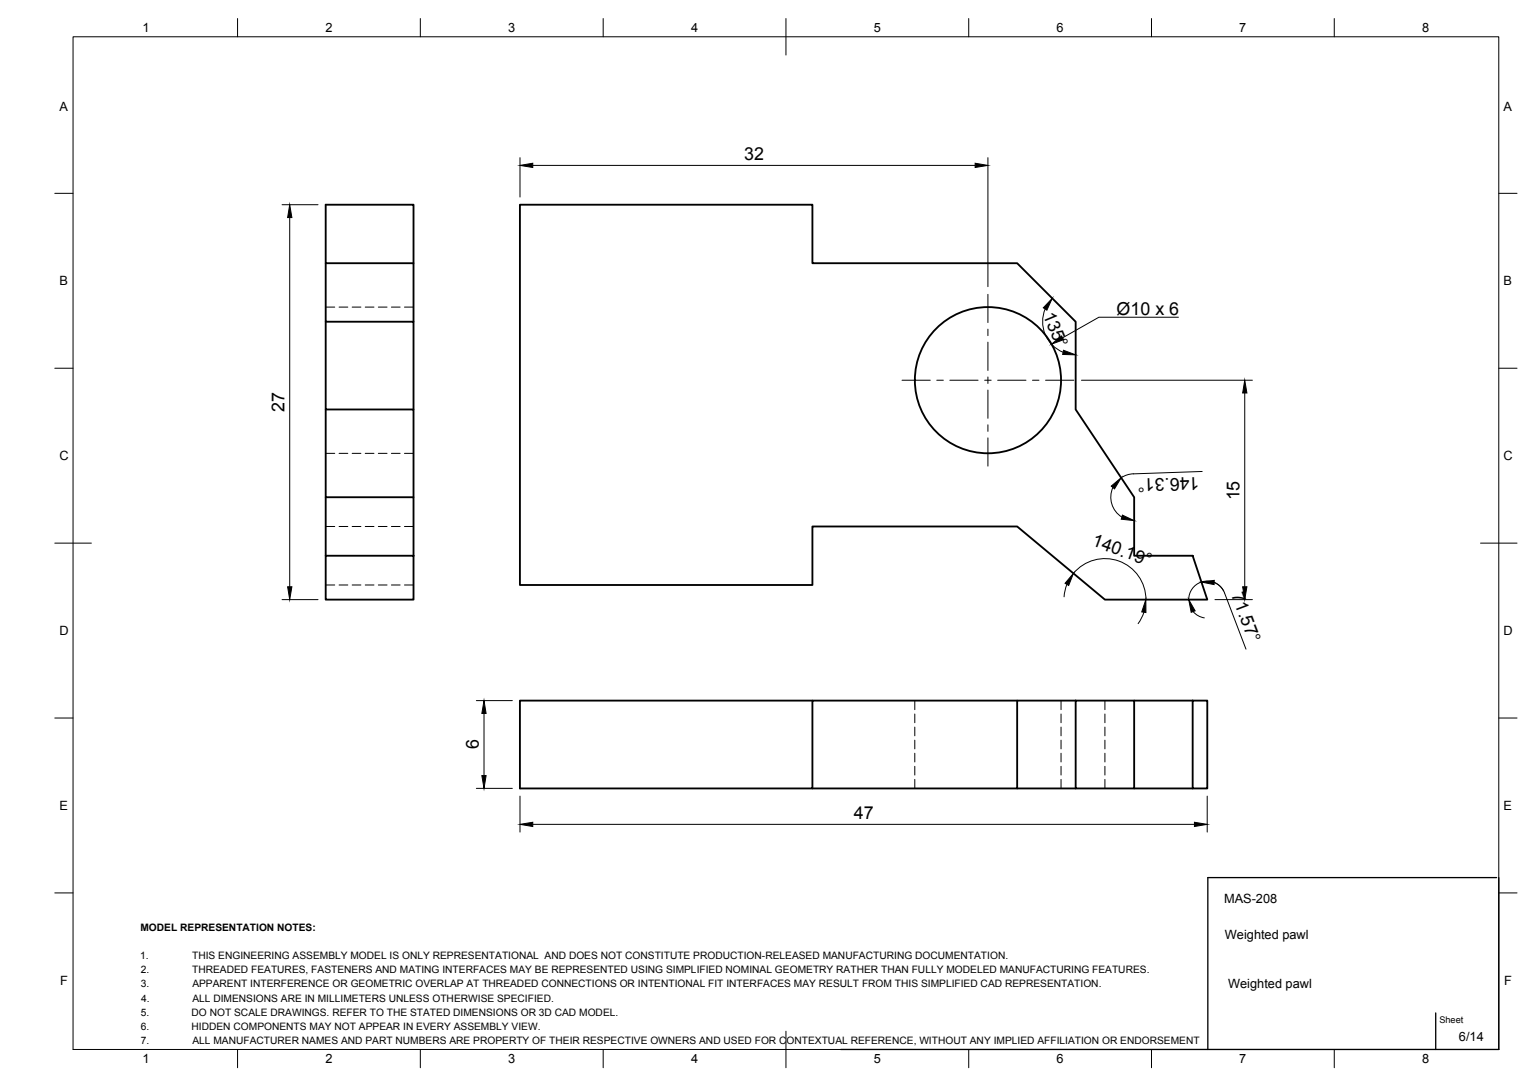
ISO-10303-21;
HEADER;
/* Generated by software containing ST-Developer
 * from STEP Tools, Inc. (www.steptools.com) 
 */

FILE_DESCRIPTION(
/* description */ ('Independent vertical20-tooth ratchet advance with repeated integral-c
ounterweight gravity pawls, swinging drive lever, bronze sleeves and f
ully retained axle stacks.18degpertooth. Native revolutes; geometric c
ycle checking rather than automatic contact/rolling dynamics. Gravity 
closing checked from actual pawl center of mass. Backplate/foot suppor
ts unit. Fits, torque, holding force, wear and life unassigned.'),
/* implementation_level */ '2;1');

FILE_NAME(
/* name */ 'Weighted pawl.step',
/* time_stamp */ '2026-11-09T06:25:53-08:00',
/* author */ (''),
/* organization */ (''),
/* preprocessor_version */ 'ST-DEVELOPER v20.2',
/* originating_system */ 'Autodesk Translation Framework v15.17.0.0',
/* authorisation */ '');

FILE_SCHEMA (('AUTOMOTIVE_DESIGN { 1 0 10303 214 3 1 1 }'));
ENDSEC;

DATA;
#10=MECHANICAL_DESIGN_GEOMETRIC_PRESENTATION_REPRESENTATION('',(#130),#4643);
#102=SHAPE_REPRESENTATION_RELATIONSHIP('SRR','None',#4707,#116);
#116=ADVANCED_BREP_SHAPE_REPRESENTATION('',(#144),#4636);
#130=STYLED_ITEM('',(#4784),#144);
#144=MANIFOLD_SOLID_BREP('Body1',#2666);
#180=FACE_BOUND('',#604,.T.);
#181=FACE_BOUND('',#606,.T.);
#273=PLANE('',#2993);
#274=PLANE('',#2994);
#275=PLANE('',#2995);
#276=PLANE('',#2996);
#277=PLANE('',#2997);
#278=PLANE('',#2998);
#279=PLANE('',#2999);
#280=PLANE('',#3000);
#281=PLANE('',#3001);
#282=PLANE('',#3002);
#283=PLANE('',#3003);
#284=PLANE('',#3004);
#285=PLANE('',#3005);
#286=PLANE('',#3006);
#287=PLANE('',#3007);
#288=PLANE('',#3008);
#289=PLANE('',#3009);
#409=FACE_OUTER_BOUND('',#587,.T.);
#410=FACE_OUTER_BOUND('',#588,.T.);
#411=FACE_OUTER_BOUND('',#589,.T.);
#412=FACE_OUTER_BOUND('',#590,.T.);
#413=FACE_OUTER_BOUND('',#591,.T.);
#414=FACE_OUTER_BOUND('',#592,.T.);
#415=FACE_OUTER_BOUND('',#593,.T.);
#416=FACE_OUTER_BOUND('',#594,.T.);
#417=FACE_OUTER_BOUND('',#595,.T.);
#418=FACE_OUTER_BOUND('',#596,.T.);
#419=FACE_OUTER_BOUND('',#597,.T.);
#420=FACE_OUTER_BOUND('',#598,.T.);
#421=FACE_OUTER_BOUND('',#599,.T.);
#422=FACE_OUTER_BOUND('',#600,.T.);
#423=FACE_OUTER_BOUND('',#601,.T.);
#424=FACE_OUTER_BOUND('',#602,.T.);
#425=FACE_OUTER_BOUND('',#603,.T.);
#426=FACE_OUTER_BOUND('',#605,.T.);
#587=EDGE_LOOP('',(#2293,#2294,#2295,#2296));
#588=EDGE_LOOP('',(#2297,#2298,#2299,#2300));
#589=EDGE_LOOP('',(#2301,#2302,#2303,#2304));
#590=EDGE_LOOP('',(#2305,#2306,#2307,#2308));
#591=EDGE_LOOP('',(#2309,#2310,#2311,#2312));
#592=EDGE_LOOP('',(#2313,#2314,#2315,#2316));
#593=EDGE_LOOP('',(#2317,#2318,#2319,#2320));
#594=EDGE_LOOP('',(#2321,#2322,#2323,#2324));
#595=EDGE_LOOP('',(#2325,#2326,#2327,#2328));
#596=EDGE_LOOP('',(#2329,#2330,#2331,#2332));
#597=EDGE_LOOP('',(#2333,#2334,#2335,#2336));
#598=EDGE_LOOP('',(#2337,#2338,#2339,#2340));
#599=EDGE_LOOP('',(#2341,#2342,#2343,#2344));
#600=EDGE_LOOP('',(#2345,#2346,#2347,#2348));
#601=EDGE_LOOP('',(#2349,#2350,#2351,#2352));
#602=EDGE_LOOP('',(#2353,#2354,#2355,#2356));
#603=EDGE_LOOP('',(#2357,#2358,#2359,#2360,#2361,#2362,#2363,#2364,#2365,
#2366,#2367,#2368,#2369,#2370,#2371));
#604=EDGE_LOOP('',(#2372));
#605=EDGE_LOOP('',(#2373,#2374,#2375,#2376,#2377,#2378,#2379,#2380,#2381,
#2382,#2383,#2384,#2385,#2386,#2387));
#606=EDGE_LOOP('',(#2388));
#841=LINE('',#4395,#1103);
#842=LINE('',#4400,#1104);
#843=LINE('',#4402,#1105);
#844=LINE('',#4404,#1106);
#845=LINE('',#4405,#1107);
#846=LINE('',#4408,#1108);
#847=LINE('',#4410,#1109);
#848=LINE('',#4411,#1110);
#849=LINE('',#4414,#1111);
#850=LINE('',#4416,#1112);
#851=LINE('',#4417,#1113);
#852=LINE('',#4420,#1114);
#853=LINE('',#4422,#1115);
#854=LINE('',#4423,#1116);
#855=LINE('',#4426,#1117);
#856=LINE('',#4428,#1118);
#857=LINE('',#4429,#1119);
#858=LINE('',#4432,#1120);
#859=LINE('',#4434,#1121);
#860=LINE('',#4435,#1122);
#861=LINE('',#4438,#1123);
#862=LINE('',#4440,#1124);
#863=LINE('',#4441,#1125);
#864=LINE('',#4444,#1126);
#865=LINE('',#4446,#1127);
#866=LINE('',#4447,#1128);
#867=LINE('',#4450,#1129);
#868=LINE('',#4452,#1130);
#869=LINE('',#4453,#1131);
#870=LINE('',#4456,#1132);
#871=LINE('',#4458,#1133);
#872=LINE('',#4459,#1134);
#873=LINE('',#4462,#1135);
#874=LINE('',#4464,#1136);
#875=LINE('',#4465,#1137);
#876=LINE('',#4468,#1138);
#877=LINE('',#4470,#1139);
#878=LINE('',#4471,#1140);
#879=LINE('',#4474,#1141);
#880=LINE('',#4476,#1142);
#881=LINE('',#4477,#1143);
#882=LINE('',#4480,#1144);
#883=LINE('',#4482,#1145);
#884=LINE('',#4483,#1146);
#885=LINE('',#4485,#1147);
#886=LINE('',#4486,#1148);
#1103=VECTOR('',#3613,5.);
#1104=VECTOR('',#3618,10.);
#1105=VECTOR('',#3619,10.);
#1106=VECTOR('',#3620,10.);
#1107=VECTOR('',#3621,10.);
#1108=VECTOR('',#3624,10.);
#1109=VECTOR('',#3625,10.);
#1110=VECTOR('',#3626,10.);
#1111=VECTOR('',#3629,10.);
#1112=VECTOR('',#3630,10.);
#1113=VECTOR('',#3631,10.);
#1114=VECTOR('',#3634,10.);
#1115=VECTOR('',#3635,10.);
#1116=VECTOR('',#3636,10.);
#1117=VECTOR('',#3639,10.);
#1118=VECTOR('',#3640,10.);
#1119=VECTOR('',#3641,10.);
#1120=VECTOR('',#3644,10.);
#1121=VECTOR('',#3645,10.);
#1122=VECTOR('',#3646,10.);
#1123=VECTOR('',#3649,10.);
#1124=VECTOR('',#3650,10.);
#1125=VECTOR('',#3651,10.);
#1126=VECTOR('',#3654,10.);
#1127=VECTOR('',#3655,10.);
#1128=VECTOR('',#3656,10.);
#1129=VECTOR('',#3659,10.);
#1130=VECTOR('',#3660,10.);
#1131=VECTOR('',#3661,10.);
#1132=VECTOR('',#3664,10.);
#1133=VECTOR('',#3665,10.);
#1134=VECTOR('',#3666,10.);
#1135=VECTOR('',#3669,10.);
#1136=VECTOR('',#3670,10.);
#1137=VECTOR('',#3671,10.);
#1138=VECTOR('',#3674,10.);
#1139=VECTOR('',#3675,10.);
#1140=VECTOR('',#3676,10.);
#1141=VECTOR('',#3679,10.);
#1142=VECTOR('',#3680,10.);
#1143=VECTOR('',#3681,10.);
#1144=VECTOR('',#3684,10.);
#1145=VECTOR('',#3685,10.);
#1146=VECTOR('',#3686,10.);
#1147=VECTOR('',#3689,10.);
#1148=VECTOR('',#3690,10.);
#1215=CIRCLE('',#2991,5.);
#1216=CIRCLE('',#2992,5.);
#1405=VERTEX_POINT('',#4392);
#1406=VERTEX_POINT('',#4394);
#1407=VERTEX_POINT('',#4398);
#1408=VERTEX_POINT('',#4399);
#1409=VERTEX_POINT('',#4401);
#1410=VERTEX_POINT('',#4403);
#1411=VERTEX_POINT('',#4407);
#1412=VERTEX_POINT('',#4409);
#1413=VERTEX_POINT('',#4413);
#1414=VERTEX_POINT('',#4415);
#1415=VERTEX_POINT('',#4419);
#1416=VERTEX_POINT('',#4421);
#1417=VERTEX_POINT('',#4425);
#1418=VERTEX_POINT('',#4427);
#1419=VERTEX_POINT('',#4431);
#1420=VERTEX_POINT('',#4433);
#1421=VERTEX_POINT('',#4437);
#1422=VERTEX_POINT('',#4439);
#1423=VERTEX_POINT('',#4443);
#1424=VERTEX_POINT('',#4445);
#1425=VERTEX_POINT('',#4449);
#1426=VERTEX_POINT('',#4451);
#1427=VERTEX_POINT('',#4455);
#1428=VERTEX_POINT('',#4457);
#1429=VERTEX_POINT('',#4461);
#1430=VERTEX_POINT('',#4463);
#1431=VERTEX_POINT('',#4467);
#1432=VERTEX_POINT('',#4469);
#1433=VERTEX_POINT('',#4473);
#1434=VERTEX_POINT('',#4475);
#1435=VERTEX_POINT('',#4479);
#1436=VERTEX_POINT('',#4481);
#1711=EDGE_CURVE('',#1405,#1405,#1215,.T.);
#1712=EDGE_CURVE('',#1405,#1406,#841,.T.);
#1713=EDGE_CURVE('',#1406,#1406,#1216,.T.);
#1714=EDGE_CURVE('',#1407,#1408,#842,.T.);
#1715=EDGE_CURVE('',#1408,#1409,#843,.T.);
#1716=EDGE_CURVE('',#1410,#1409,#844,.T.);
#1717=EDGE_CURVE('',#1407,#1410,#845,.T.);
#1718=EDGE_CURVE('',#1411,#1407,#846,.T.);
#1719=EDGE_CURVE('',#1412,#1410,#847,.T.);
#1720=EDGE_CURVE('',#1411,#1412,#848,.T.);
#1721=EDGE_CURVE('',#1413,#1411,#849,.T.);
#1722=EDGE_CURVE('',#1414,#1412,#850,.T.);
#1723=EDGE_CURVE('',#1413,#1414,#851,.T.);
#1724=EDGE_CURVE('',#1415,#1413,#852,.T.);
#1725=EDGE_CURVE('',#1416,#1414,#853,.T.);
#1726=EDGE_CURVE('',#1415,#1416,#854,.T.);
#1727=EDGE_CURVE('',#1417,#1415,#855,.T.);
#1728=EDGE_CURVE('',#1418,#1416,#856,.T.);
#1729=EDGE_CURVE('',#1417,#1418,#857,.T.);
#1730=EDGE_CURVE('',#1419,#1417,#858,.T.);
#1731=EDGE_CURVE('',#1420,#1418,#859,.T.);
#1732=EDGE_CURVE('',#1419,#1420,#860,.T.);
#1733=EDGE_CURVE('',#1421,#1419,#861,.T.);
#1734=EDGE_CURVE('',#1422,#1420,#862,.T.);
#1735=EDGE_CURVE('',#1421,#1422,#863,.T.);
#1736=EDGE_CURVE('',#1423,#1421,#864,.T.);
#1737=EDGE_CURVE('',#1424,#1422,#865,.T.);
#1738=EDGE_CURVE('',#1423,#1424,#866,.T.);
#1739=EDGE_CURVE('',#1425,#1423,#867,.T.);
#1740=EDGE_CURVE('',#1426,#1424,#868,.T.);
#1741=EDGE_CURVE('',#1425,#1426,#869,.T.);
#1742=EDGE_CURVE('',#1427,#1425,#870,.T.);
#1743=EDGE_CURVE('',#1428,#1426,#871,.T.);
#1744=EDGE_CURVE('',#1427,#1428,#872,.T.);
#1745=EDGE_CURVE('',#1429,#1427,#873,.T.);
#1746=EDGE_CURVE('',#1430,#1428,#874,.T.);
#1747=EDGE_CURVE('',#1429,#1430,#875,.T.);
#1748=EDGE_CURVE('',#1431,#1429,#876,.T.);
#1749=EDGE_CURVE('',#1432,#1430,#877,.T.);
#1750=EDGE_CURVE('',#1431,#1432,#878,.T.);
#1751=EDGE_CURVE('',#1433,#1431,#879,.T.);
#1752=EDGE_CURVE('',#1434,#1432,#880,.T.);
#1753=EDGE_CURVE('',#1433,#1434,#881,.T.);
#1754=EDGE_CURVE('',#1435,#1433,#882,.T.);
#1755=EDGE_CURVE('',#1436,#1434,#883,.T.);
#1756=EDGE_CURVE('',#1435,#1436,#884,.T.);
#1757=EDGE_CURVE('',#1408,#1435,#885,.T.);
#1758=EDGE_CURVE('',#1409,#1436,#886,.T.);
#2293=ORIENTED_EDGE('',*,*,#1711,.F.);
#2294=ORIENTED_EDGE('',*,*,#1712,.T.);
#2295=ORIENTED_EDGE('',*,*,#1713,.F.);
#2296=ORIENTED_EDGE('',*,*,#1712,.F.);
#2297=ORIENTED_EDGE('',*,*,#1714,.T.);
#2298=ORIENTED_EDGE('',*,*,#1715,.T.);
#2299=ORIENTED_EDGE('',*,*,#1716,.F.);
#2300=ORIENTED_EDGE('',*,*,#1717,.F.);
#2301=ORIENTED_EDGE('',*,*,#1718,.T.);
#2302=ORIENTED_EDGE('',*,*,#1717,.T.);
#2303=ORIENTED_EDGE('',*,*,#1719,.F.);
#2304=ORIENTED_EDGE('',*,*,#1720,.F.);
#2305=ORIENTED_EDGE('',*,*,#1721,.T.);
#2306=ORIENTED_EDGE('',*,*,#1720,.T.);
#2307=ORIENTED_EDGE('',*,*,#1722,.F.);
#2308=ORIENTED_EDGE('',*,*,#1723,.F.);
#2309=ORIENTED_EDGE('',*,*,#1724,.T.);
#2310=ORIENTED_EDGE('',*,*,#1723,.T.);
#2311=ORIENTED_EDGE('',*,*,#1725,.F.);
#2312=ORIENTED_EDGE('',*,*,#1726,.F.);
#2313=ORIENTED_EDGE('',*,*,#1727,.T.);
#2314=ORIENTED_EDGE('',*,*,#1726,.T.);
#2315=ORIENTED_EDGE('',*,*,#1728,.F.);
#2316=ORIENTED_EDGE('',*,*,#1729,.F.);
#2317=ORIENTED_EDGE('',*,*,#1730,.T.);
#2318=ORIENTED_EDGE('',*,*,#1729,.T.);
#2319=ORIENTED_EDGE('',*,*,#1731,.F.);
#2320=ORIENTED_EDGE('',*,*,#1732,.F.);
#2321=ORIENTED_EDGE('',*,*,#1733,.T.);
#2322=ORIENTED_EDGE('',*,*,#1732,.T.);
#2323=ORIENTED_EDGE('',*,*,#1734,.F.);
#2324=ORIENTED_EDGE('',*,*,#1735,.F.);
#2325=ORIENTED_EDGE('',*,*,#1736,.T.);
#2326=ORIENTED_EDGE('',*,*,#1735,.T.);
#2327=ORIENTED_EDGE('',*,*,#1737,.F.);
#2328=ORIENTED_EDGE('',*,*,#1738,.F.);
#2329=ORIENTED_EDGE('',*,*,#1739,.T.);
#2330=ORIENTED_EDGE('',*,*,#1738,.T.);
#2331=ORIENTED_EDGE('',*,*,#1740,.F.);
#2332=ORIENTED_EDGE('',*,*,#1741,.F.);
#2333=ORIENTED_EDGE('',*,*,#1742,.T.);
#2334=ORIENTED_EDGE('',*,*,#1741,.T.);
#2335=ORIENTED_EDGE('',*,*,#1743,.F.);
#2336=ORIENTED_EDGE('',*,*,#1744,.F.);
#2337=ORIENTED_EDGE('',*,*,#1745,.T.);
#2338=ORIENTED_EDGE('',*,*,#1744,.T.);
#2339=ORIENTED_EDGE('',*,*,#1746,.F.);
#2340=ORIENTED_EDGE('',*,*,#1747,.F.);
#2341=ORIENTED_EDGE('',*,*,#1748,.T.);
#2342=ORIENTED_EDGE('',*,*,#1747,.T.);
#2343=ORIENTED_EDGE('',*,*,#1749,.F.);
#2344=ORIENTED_EDGE('',*,*,#1750,.F.);
#2345=ORIENTED_EDGE('',*,*,#1751,.T.);
#2346=ORIENTED_EDGE('',*,*,#1750,.T.);
#2347=ORIENTED_EDGE('',*,*,#1752,.F.);
#2348=ORIENTED_EDGE('',*,*,#1753,.F.);
#2349=ORIENTED_EDGE('',*,*,#1754,.T.);
#2350=ORIENTED_EDGE('',*,*,#1753,.T.);
#2351=ORIENTED_EDGE('',*,*,#1755,.F.);
#2352=ORIENTED_EDGE('',*,*,#1756,.F.);
#2353=ORIENTED_EDGE('',*,*,#1757,.T.);
#2354=ORIENTED_EDGE('',*,*,#1756,.T.);
#2355=ORIENTED_EDGE('',*,*,#1758,.F.);
#2356=ORIENTED_EDGE('',*,*,#1715,.F.);
#2357=ORIENTED_EDGE('',*,*,#1758,.T.);
#2358=ORIENTED_EDGE('',*,*,#1755,.T.);
#2359=ORIENTED_EDGE('',*,*,#1752,.T.);
#2360=ORIENTED_EDGE('',*,*,#1749,.T.);
#2361=ORIENTED_EDGE('',*,*,#1746,.T.);
#2362=ORIENTED_EDGE('',*,*,#1743,.T.);
#2363=ORIENTED_EDGE('',*,*,#1740,.T.);
#2364=ORIENTED_EDGE('',*,*,#1737,.T.);
#2365=ORIENTED_EDGE('',*,*,#1734,.T.);
#2366=ORIENTED_EDGE('',*,*,#1731,.T.);
#2367=ORIENTED_EDGE('',*,*,#1728,.T.);
#2368=ORIENTED_EDGE('',*,*,#1725,.T.);
#2369=ORIENTED_EDGE('',*,*,#1722,.T.);
#2370=ORIENTED_EDGE('',*,*,#1719,.T.);
#2371=ORIENTED_EDGE('',*,*,#1716,.T.);
#2372=ORIENTED_EDGE('',*,*,#1711,.T.);
#2373=ORIENTED_EDGE('',*,*,#1757,.F.);
#2374=ORIENTED_EDGE('',*,*,#1714,.F.);
#2375=ORIENTED_EDGE('',*,*,#1718,.F.);
#2376=ORIENTED_EDGE('',*,*,#1721,.F.);
#2377=ORIENTED_EDGE('',*,*,#1724,.F.);
#2378=ORIENTED_EDGE('',*,*,#1727,.F.);
#2379=ORIENTED_EDGE('',*,*,#1730,.F.);
#2380=ORIENTED_EDGE('',*,*,#1733,.F.);
#2381=ORIENTED_EDGE('',*,*,#1736,.F.);
#2382=ORIENTED_EDGE('',*,*,#1739,.F.);
#2383=ORIENTED_EDGE('',*,*,#1742,.F.);
#2384=ORIENTED_EDGE('',*,*,#1745,.F.);
#2385=ORIENTED_EDGE('',*,*,#1748,.F.);
#2386=ORIENTED_EDGE('',*,*,#1751,.F.);
#2387=ORIENTED_EDGE('',*,*,#1754,.F.);
#2388=ORIENTED_EDGE('',*,*,#1713,.T.);
#2497=CYLINDRICAL_SURFACE('',#2990,5.);
#2615=ADVANCED_FACE('',(#409),#2497,.F.);
#2616=ADVANCED_FACE('',(#410),#273,.T.);
#2617=ADVANCED_FACE('',(#411),#274,.T.);
#2618=ADVANCED_FACE('',(#412),#275,.T.);
#2619=ADVANCED_FACE('',(#413),#276,.T.);
#2620=ADVANCED_FACE('',(#414),#277,.T.);
#2621=ADVANCED_FACE('',(#415),#278,.T.);
#2622=ADVANCED_FACE('',(#416),#279,.T.);
#2623=ADVANCED_FACE('',(#417),#280,.T.);
#2624=ADVANCED_FACE('',(#418),#281,.T.);
#2625=ADVANCED_FACE('',(#419),#282,.T.);
#2626=ADVANCED_FACE('',(#420),#283,.T.);
#2627=ADVANCED_FACE('',(#421),#284,.T.);
#2628=ADVANCED_FACE('',(#422),#285,.T.);
#2629=ADVANCED_FACE('',(#423),#286,.T.);
#2630=ADVANCED_FACE('',(#424),#287,.T.);
#2631=ADVANCED_FACE('',(#425,#180),#288,.T.);
#2632=ADVANCED_FACE('',(#426,#181),#289,.F.);
#2666=CLOSED_SHELL('',(#2615,#2616,#2617,#2618,#2619,#2620,#2621,#2622,
#2623,#2624,#2625,#2626,#2627,#2628,#2629,#2630,#2631,#2632));
#2989=AXIS2_PLACEMENT_3D('',#4390,#3607,#3608);
#2990=AXIS2_PLACEMENT_3D('',#4391,#3609,#3610);
#2991=AXIS2_PLACEMENT_3D('',#4393,#3611,#3612);
#2992=AXIS2_PLACEMENT_3D('',#4396,#3614,#3615);
#2993=AXIS2_PLACEMENT_3D('',#4397,#3616,#3617);
#2994=AXIS2_PLACEMENT_3D('',#4406,#3622,#3623);
#2995=AXIS2_PLACEMENT_3D('',#4412,#3627,#3628);
#2996=AXIS2_PLACEMENT_3D('',#4418,#3632,#3633);
#2997=AXIS2_PLACEMENT_3D('',#4424,#3637,#3638);
#2998=AXIS2_PLACEMENT_3D('',#4430,#3642,#3643);
#2999=AXIS2_PLACEMENT_3D('',#4436,#3647,#3648);
#3000=AXIS2_PLACEMENT_3D('',#4442,#3652,#3653);
#3001=AXIS2_PLACEMENT_3D('',#4448,#3657,#3658);
#3002=AXIS2_PLACEMENT_3D('',#4454,#3662,#3663);
#3003=AXIS2_PLACEMENT_3D('',#4460,#3667,#3668);
#3004=AXIS2_PLACEMENT_3D('',#4466,#3672,#3673);
#3005=AXIS2_PLACEMENT_3D('',#4472,#3677,#3678);
#3006=AXIS2_PLACEMENT_3D('',#4478,#3682,#3683);
#3007=AXIS2_PLACEMENT_3D('',#4484,#3687,#3688);
#3008=AXIS2_PLACEMENT_3D('',#4487,#3691,#3692);
#3009=AXIS2_PLACEMENT_3D('',#4488,#3693,#3694);
#3607=DIRECTION('axis',(0.,0.,1.));
#3608=DIRECTION('refdir',(1.,0.,0.));
#3609=DIRECTION('center_axis',(0.,0.,-1.));
#3610=DIRECTION('ref_axis',(1.,0.,0.));
#3611=DIRECTION('center_axis',(0.,0.,-1.));
#3612=DIRECTION('ref_axis',(1.,0.,0.));
#3613=DIRECTION('',(0.,0.,-1.));
#3614=DIRECTION('center_axis',(0.,0.,1.));
#3615=DIRECTION('ref_axis',(1.,0.,0.));
#3616=DIRECTION('center_axis',(-1.,0.,0.));
#3617=DIRECTION('ref_axis',(0.,-1.,0.));
#3618=DIRECTION('',(0.,-1.,0.));
#3619=DIRECTION('',(0.,0.,1.));
#3620=DIRECTION('',(0.,-1.,0.));
#3621=DIRECTION('',(0.,0.,1.));
#3622=DIRECTION('center_axis',(-0.832050294337843,0.554700196225229,0.));
#3623=DIRECTION('ref_axis',(-0.554700196225229,-0.832050294337843,0.));
#3624=DIRECTION('',(-0.554700196225229,-0.832050294337843,0.));
#3625=DIRECTION('',(-0.554700196225229,-0.832050294337843,0.));
#3626=DIRECTION('',(0.,0.,1.));
#3627=DIRECTION('center_axis',(-1.,0.,0.));
#3628=DIRECTION('ref_axis',(0.,-1.,0.));
#3629=DIRECTION('',(0.,-1.,0.));
#3630=DIRECTION('',(0.,-1.,0.));
#3631=DIRECTION('',(0.,0.,1.));
#3632=DIRECTION('center_axis',(-0.707106781186548,0.707106781186547,0.));
#3633=DIRECTION('ref_axis',(-0.707106781186547,-0.707106781186548,0.));
#3634=DIRECTION('',(-0.707106781186547,-0.707106781186548,0.));
#3635=DIRECTION('',(-0.707106781186547,-0.707106781186548,0.));
#3636=DIRECTION('',(0.,0.,1.));
#3637=DIRECTION('center_axis',(0.,1.,0.));
#3638=DIRECTION('ref_axis',(-1.,0.,0.));
#3639=DIRECTION('',(-1.,0.,0.));
#3640=DIRECTION('',(-1.,0.,0.));
#3641=DIRECTION('',(0.,0.,1.));
#3642=DIRECTION('center_axis',(-1.,0.,0.));
#3643=DIRECTION('ref_axis',(0.,-1.,0.));
#3644=DIRECTION('',(0.,-1.,0.));
#3645=DIRECTION('',(0.,-1.,0.));
#3646=DIRECTION('',(0.,0.,1.));
#3647=DIRECTION('center_axis',(0.,1.,0.));
#3648=DIRECTION('ref_axis',(-1.,0.,0.));
#3649=DIRECTION('',(-1.,0.,0.));
#3650=DIRECTION('',(-1.,0.,0.));
#3651=DIRECTION('',(0.,0.,1.));
#3652=DIRECTION('center_axis',(1.,0.,0.));
#3653=DIRECTION('ref_axis',(0.,1.,0.));
#3654=DIRECTION('',(0.,1.,0.));
#3655=DIRECTION('',(0.,1.,0.));
#3656=DIRECTION('',(0.,0.,1.));
#3657=DIRECTION('center_axis',(0.,-1.,0.));
#3658=DIRECTION('ref_axis',(1.,0.,0.));
#3659=DIRECTION('',(1.,0.,0.));
#3660=DIRECTION('',(1.,0.,0.));
#3661=DIRECTION('',(0.,0.,1.));
#3662=DIRECTION('center_axis',(-1.,0.,0.));
#3663=DIRECTION('ref_axis',(0.,-1.,0.));
#3664=DIRECTION('',(0.,-1.,0.));
#3665=DIRECTION('',(0.,-1.,0.));
#3666=DIRECTION('',(0.,0.,1.));
#3667=DIRECTION('center_axis',(0.,-1.,0.));
#3668=DIRECTION('ref_axis',(1.,0.,0.));
#3669=DIRECTION('',(1.,0.,0.));
#3670=DIRECTION('',(1.,0.,0.));
#3671=DIRECTION('',(0.,0.,1.));
#3672=DIRECTION('center_axis',(0.64018439966448,-0.768221279597376,0.));
#3673=DIRECTION('ref_axis',(0.768221279597376,0.64018439966448,0.));
#3674=DIRECTION('',(0.768221279597376,0.64018439966448,0.));
#3675=DIRECTION('',(0.768221279597376,0.64018439966448,0.));
#3676=DIRECTION('',(0.,0.,1.));
#3677=DIRECTION('center_axis',(0.,-1.,0.));
#3678=DIRECTION('ref_axis',(1.,0.,0.));
#3679=DIRECTION('',(1.,0.,0.));
#3680=DIRECTION('',(1.,0.,0.));
#3681=DIRECTION('',(0.,0.,1.));
#3682=DIRECTION('center_axis',(-0.948683298050514,0.316227766016838,0.));
#3683=DIRECTION('ref_axis',(-0.316227766016838,-0.948683298050514,0.));
#3684=DIRECTION('',(-0.316227766016838,-0.948683298050514,0.));
#3685=DIRECTION('',(-0.316227766016838,-0.948683298050514,0.));
#3686=DIRECTION('',(0.,0.,1.));
#3687=DIRECTION('center_axis',(0.,1.,0.));
#3688=DIRECTION('ref_axis',(-1.,0.,0.));
#3689=DIRECTION('',(-1.,0.,0.));
#3690=DIRECTION('',(-1.,0.,0.));
#3691=DIRECTION('center_axis',(0.,0.,1.));
#3692=DIRECTION('ref_axis',(1.,0.,0.));
#3693=DIRECTION('center_axis',(0.,0.,1.));
#3694=DIRECTION('ref_axis',(1.,0.,0.));
#4390=CARTESIAN_POINT('',(0.,0.,0.));
#4391=CARTESIAN_POINT('Origin',(50.,12.,3.));
#4392=CARTESIAN_POINT('',(45.,12.,6.));
#4393=CARTESIAN_POINT('Origin',(50.,12.,6.));
#4394=CARTESIAN_POINT('',(45.,12.,0.));
#4395=CARTESIAN_POINT('',(45.,12.,3.));
#4396=CARTESIAN_POINT('Origin',(50.,12.,0.));
#4397=CARTESIAN_POINT('Origin',(40.,4.,0.));
#4398=CARTESIAN_POINT('',(40.,4.,0.));
#4399=CARTESIAN_POINT('',(40.,0.,0.));
#4400=CARTESIAN_POINT('',(40.,4.,0.));
#4401=CARTESIAN_POINT('',(40.,0.,6.));
#4402=CARTESIAN_POINT('',(40.,0.,0.));
#4403=CARTESIAN_POINT('',(40.,4.,6.));
#4404=CARTESIAN_POINT('',(40.,4.,6.));
#4405=CARTESIAN_POINT('',(40.,4.,0.));
#4406=CARTESIAN_POINT('Origin',(44.,10.,0.));
#4407=CARTESIAN_POINT('',(44.,10.,0.));
#4408=CARTESIAN_POINT('',(44.,10.,0.));
#4409=CARTESIAN_POINT('',(44.,10.,6.));
#4410=CARTESIAN_POINT('',(44.,10.,6.));
#4411=CARTESIAN_POINT('',(44.,10.,0.));
#4412=CARTESIAN_POINT('Origin',(44.,16.,0.));
#4413=CARTESIAN_POINT('',(44.,16.,0.));
#4414=CARTESIAN_POINT('',(44.,16.,0.));
#4415=CARTESIAN_POINT('',(44.,16.,6.));
#4416=CARTESIAN_POINT('',(44.,16.,6.));
#4417=CARTESIAN_POINT('',(44.,16.,0.));
#4418=CARTESIAN_POINT('Origin',(48.,20.,0.));
#4419=CARTESIAN_POINT('',(48.,20.,0.));
#4420=CARTESIAN_POINT('',(48.,20.,0.));
#4421=CARTESIAN_POINT('',(48.,20.,6.));
#4422=CARTESIAN_POINT('',(48.,20.,6.));
#4423=CARTESIAN_POINT('',(48.,20.,0.));
#4424=CARTESIAN_POINT('Origin',(62.,20.,0.));
#4425=CARTESIAN_POINT('',(62.,20.,0.));
#4426=CARTESIAN_POINT('',(62.,20.,0.));
#4427=CARTESIAN_POINT('',(62.,20.,6.));
#4428=CARTESIAN_POINT('',(62.,20.,6.));
#4429=CARTESIAN_POINT('',(62.,20.,0.));
#4430=CARTESIAN_POINT('Origin',(62.,24.,0.));
#4431=CARTESIAN_POINT('',(62.,24.,0.));
#4432=CARTESIAN_POINT('',(62.,24.,0.));
#4433=CARTESIAN_POINT('',(62.,24.,6.));
#4434=CARTESIAN_POINT('',(62.,24.,6.));
#4435=CARTESIAN_POINT('',(62.,24.,0.));
#4436=CARTESIAN_POINT('Origin',(82.,24.,0.));
#4437=CARTESIAN_POINT('',(82.,24.,0.));
#4438=CARTESIAN_POINT('',(82.,24.,0.));
#4439=CARTESIAN_POINT('',(82.,24.,6.));
#4440=CARTESIAN_POINT('',(82.,24.,6.));
#4441=CARTESIAN_POINT('',(82.,24.,0.));
#4442=CARTESIAN_POINT('Origin',(82.,-2.,0.));
#4443=CARTESIAN_POINT('',(82.,-2.,0.));
#4444=CARTESIAN_POINT('',(82.,-2.,0.));
#4445=CARTESIAN_POINT('',(82.,-2.,6.));
#4446=CARTESIAN_POINT('',(82.,-2.,6.));
#4447=CARTESIAN_POINT('',(82.,-2.,0.));
#4448=CARTESIAN_POINT('Origin',(62.,-2.,0.));
#4449=CARTESIAN_POINT('',(62.,-2.,0.));
#4450=CARTESIAN_POINT('',(62.,-2.,0.));
#4451=CARTESIAN_POINT('',(62.,-2.,6.));
#4452=CARTESIAN_POINT('',(62.,-2.,6.));
#4453=CARTESIAN_POINT('',(62.,-2.,0.));
#4454=CARTESIAN_POINT('Origin',(62.,2.,0.));
#4455=CARTESIAN_POINT('',(62.,2.,0.));
#4456=CARTESIAN_POINT('',(62.,2.,0.));
#4457=CARTESIAN_POINT('',(62.,2.,6.));
#4458=CARTESIAN_POINT('',(62.,2.,6.));
#4459=CARTESIAN_POINT('',(62.,2.,0.));
#4460=CARTESIAN_POINT('Origin',(48.,2.,0.));
#4461=CARTESIAN_POINT('',(48.,2.,0.));
#4462=CARTESIAN_POINT('',(48.,2.,0.));
#4463=CARTESIAN_POINT('',(48.,2.,6.));
#4464=CARTESIAN_POINT('',(48.,2.,6.));
#4465=CARTESIAN_POINT('',(48.,2.,0.));
#4466=CARTESIAN_POINT('Origin',(42.,-3.,0.));
#4467=CARTESIAN_POINT('',(42.,-3.,0.));
#4468=CARTESIAN_POINT('',(42.,-3.,0.));
#4469=CARTESIAN_POINT('',(42.,-3.,6.));
#4470=CARTESIAN_POINT('',(42.,-3.,6.));
#4471=CARTESIAN_POINT('',(42.,-3.,0.));
#4472=CARTESIAN_POINT('Origin',(35.,-3.,0.));
#4473=CARTESIAN_POINT('',(35.,-3.,0.));
#4474=CARTESIAN_POINT('',(35.,-3.,0.));
#4475=CARTESIAN_POINT('',(35.,-3.,6.));
#4476=CARTESIAN_POINT('',(35.,-3.,6.));
#4477=CARTESIAN_POINT('',(35.,-3.,0.));
#4478=CARTESIAN_POINT('Origin',(36.,0.,0.));
#4479=CARTESIAN_POINT('',(36.,0.,0.));
#4480=CARTESIAN_POINT('',(36.,0.,0.));
#4481=CARTESIAN_POINT('',(36.,0.,6.));
#4482=CARTESIAN_POINT('',(36.,0.,6.));
#4483=CARTESIAN_POINT('',(36.,0.,0.));
#4484=CARTESIAN_POINT('Origin',(40.,0.,0.));
#4485=CARTESIAN_POINT('',(40.,0.,0.));
#4486=CARTESIAN_POINT('',(40.,0.,6.));
#4487=CARTESIAN_POINT('Origin',(58.5,10.5,6.));
#4488=CARTESIAN_POINT('Origin',(58.5,10.5,0.));
#4620=UNCERTAINTY_MEASURE_WITH_UNIT(LENGTH_MEASURE(0.01),#4644,
'DISTANCE_ACCURACY_VALUE',
'Maximum model space distance between geometric entities at asserted c
onnectivities');
#4627=UNCERTAINTY_MEASURE_WITH_UNIT(LENGTH_MEASURE(0.01),#4644,
'DISTANCE_ACCURACY_VALUE',
'Maximum model space distance between geometric entities at asserted c
onnectivities');
#4636=(
GEOMETRIC_REPRESENTATION_CONTEXT(3)
GLOBAL_UNCERTAINTY_ASSIGNED_CONTEXT((#4620))
GLOBAL_UNIT_ASSIGNED_CONTEXT((#4644,#4646,#4647))
REPRESENTATION_CONTEXT('','3D')
);
#4643=(
GEOMETRIC_REPRESENTATION_CONTEXT(3)
GLOBAL_UNCERTAINTY_ASSIGNED_CONTEXT((#4627))
GLOBAL_UNIT_ASSIGNED_CONTEXT((#4644,#4646,#4647))
REPRESENTATION_CONTEXT('','3D')
);
#4644=(
LENGTH_UNIT()
NAMED_UNIT(*)
SI_UNIT(.MILLI.,.METRE.)
);
#4646=(
NAMED_UNIT(*)
PLANE_ANGLE_UNIT()
SI_UNIT($,.RADIAN.)
);
#4647=(
NAMED_UNIT(*)
SI_UNIT($,.STERADIAN.)
SOLID_ANGLE_UNIT()
);
#4656=SHAPE_DEFINITION_REPRESENTATION(#4671,#4707);
#4671=PRODUCT_DEFINITION_SHAPE('',$,#4723);
#4707=SHAPE_REPRESENTATION('',(#2989),#4636);
#4714=PRODUCT_DEFINITION_CONTEXT('part definition',#4761,'design');
#4723=PRODUCT_DEFINITION('Weighted pawl','Weighted pawl',#4738,#4714);
#4738=PRODUCT_DEFINITION_FORMATION('',$,#4771);
#4761=APPLICATION_CONTEXT(
'Core Data for Automotive Mechanical Design Process');
#4762=PRODUCT_CONTEXT('part definition',#4761,'mechanical');
#4771=PRODUCT('Weighted pawl','Weighted pawl',$,(#4762));
#4784=PRESENTATION_STYLE_ASSIGNMENT((#4793));
#4793=SURFACE_STYLE_USAGE(.BOTH.,#4802);
#4802=SURFACE_SIDE_STYLE('',(#4811));
#4811=SURFACE_STYLE_FILL_AREA(#4820);
#4820=FILL_AREA_STYLE('Sky blue',(#4829));
#4829=FILL_AREA_STYLE_COLOUR('Sky blue',#4838);
#4838=COLOUR_RGB('Sky blue',0.317647058823529,0.686274509803922,0.890196078431372);
ENDSEC;
END-ISO-10303-21;
